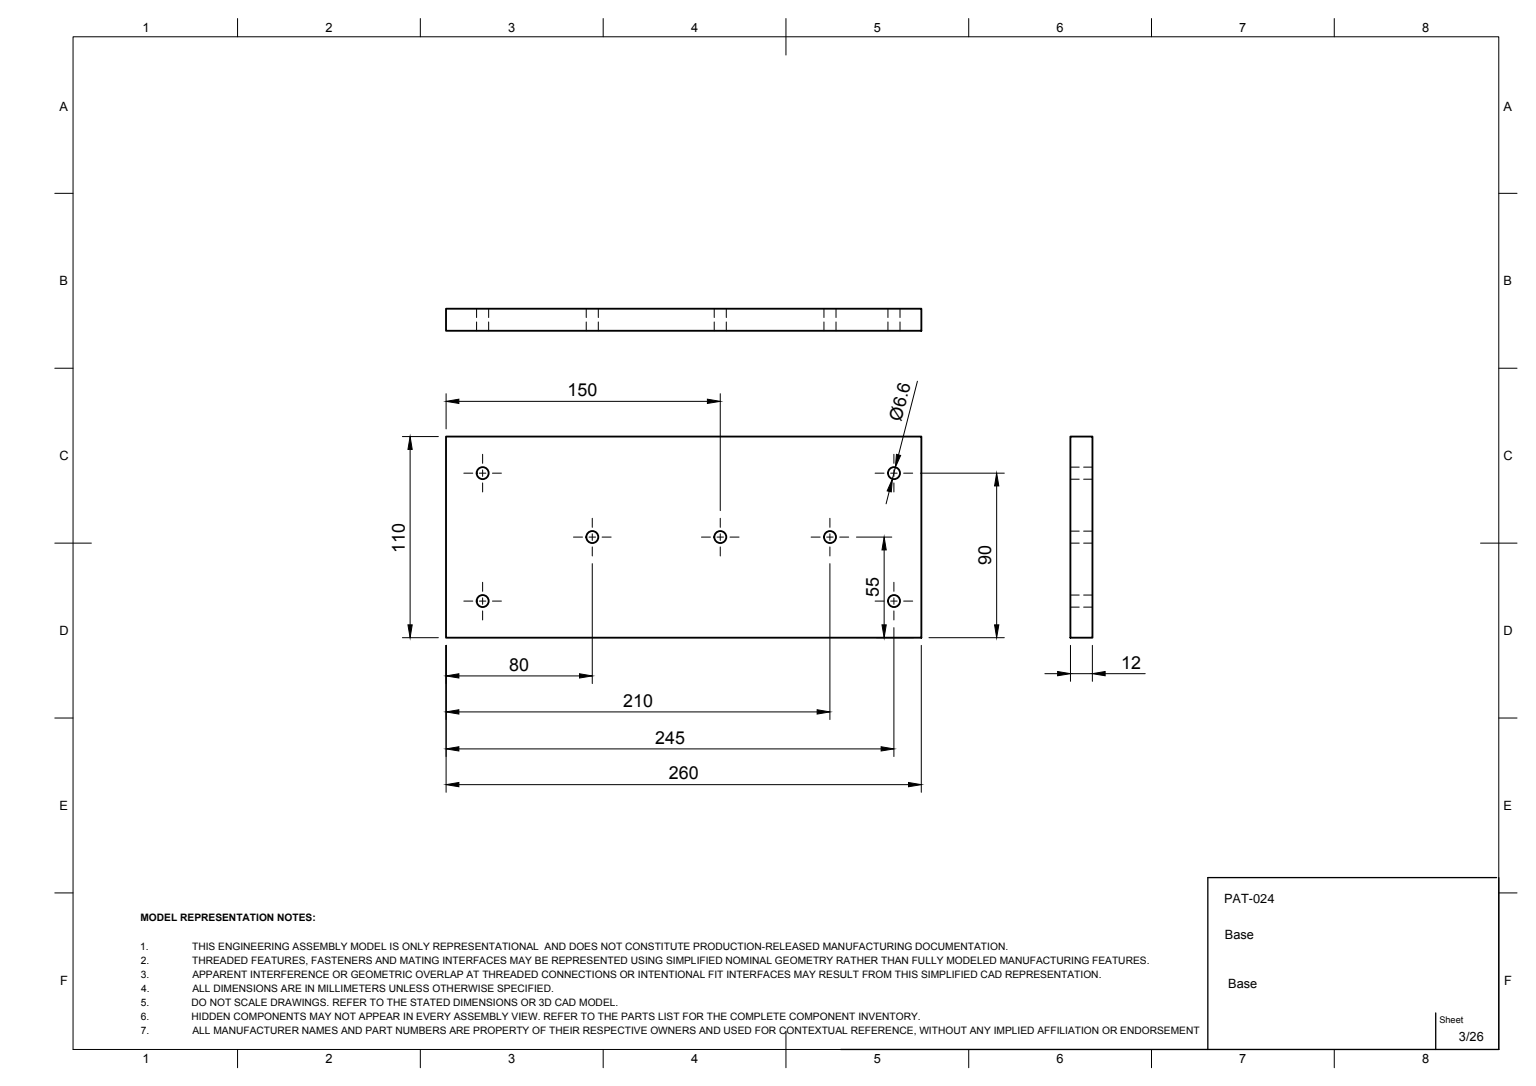
ISO-10303-21;
HEADER;
/* Generated by software containing ST-Developer
 * from STEP Tools, Inc. (www.steptools.com) 
 */

FILE_DESCRIPTION(
/* description */ ('Compact handwheel screw vise'),
/* implementation_level */ '2;1');

FILE_NAME(
/* name */ 'Base.step',
/* time_stamp */ '2026-10-29T16:08:22-07:00',
/* author */ (''),
/* organization */ (''),
/* preprocessor_version */ 'ST-DEVELOPER v20.2',
/* originating_system */ 'Autodesk Translation Framework v15.17.0.0',
/* authorisation */ '');

FILE_SCHEMA (('AUTOMOTIVE_DESIGN { 1 0 10303 214 3 1 1 }'));
ENDSEC;

DATA;
#10=MECHANICAL_DESIGN_GEOMETRIC_PRESENTATION_REPRESENTATION('',(#644),#25074);
#588=SHAPE_REPRESENTATION_RELATIONSHIP('SRR','None',#25196,#616);
#616=ADVANCED_BREP_SHAPE_REPRESENTATION('',(#680),#25043);
#644=STYLED_ITEM('',(#25418),#680);
#680=MANIFOLD_SOLID_BREP('Body1',#8052);
#712=FACE_BOUND('',#1494,.T.);
#713=FACE_BOUND('',#1495,.T.);
#714=FACE_BOUND('',#1496,.T.);
#715=FACE_BOUND('',#1497,.T.);
#716=FACE_BOUND('',#1498,.T.);
#717=FACE_BOUND('',#1499,.T.);
#718=FACE_BOUND('',#1500,.T.);
#719=FACE_BOUND('',#1502,.T.);
#720=FACE_BOUND('',#1503,.T.);
#721=FACE_BOUND('',#1504,.T.);
#722=FACE_BOUND('',#1505,.T.);
#723=FACE_BOUND('',#1506,.T.);
#724=FACE_BOUND('',#1507,.T.);
#725=FACE_BOUND('',#1508,.T.);
#822=PLANE('',#8425);
#823=PLANE('',#8426);
#824=PLANE('',#8427);
#825=PLANE('',#8428);
#826=PLANE('',#8429);
#827=PLANE('',#8430);
#1012=FACE_OUTER_BOUND('',#1482,.T.);
#1013=FACE_OUTER_BOUND('',#1483,.T.);
#1014=FACE_OUTER_BOUND('',#1484,.T.);
#1015=FACE_OUTER_BOUND('',#1485,.T.);
#1016=FACE_OUTER_BOUND('',#1486,.T.);
#1017=FACE_OUTER_BOUND('',#1487,.T.);
#1018=FACE_OUTER_BOUND('',#1488,.T.);
#1019=FACE_OUTER_BOUND('',#1489,.T.);
#1020=FACE_OUTER_BOUND('',#1490,.T.);
#1021=FACE_OUTER_BOUND('',#1491,.T.);
#1022=FACE_OUTER_BOUND('',#1492,.T.);
#1023=FACE_OUTER_BOUND('',#1493,.T.);
#1024=FACE_OUTER_BOUND('',#1501,.T.);
#1482=EDGE_LOOP('',(#5159,#5160,#5161,#5162));
#1483=EDGE_LOOP('',(#5163,#5164,#5165,#5166));
#1484=EDGE_LOOP('',(#5167,#5168,#5169,#5170));
#1485=EDGE_LOOP('',(#5171,#5172,#5173,#5174));
#1486=EDGE_LOOP('',(#5175,#5176,#5177,#5178));
#1487=EDGE_LOOP('',(#5179,#5180,#5181,#5182));
#1488=EDGE_LOOP('',(#5183,#5184,#5185,#5186));
#1489=EDGE_LOOP('',(#5187,#5188,#5189,#5190));
#1490=EDGE_LOOP('',(#5191,#5192,#5193,#5194));
#1491=EDGE_LOOP('',(#5195,#5196,#5197,#5198));
#1492=EDGE_LOOP('',(#5199,#5200,#5201,#5202));
#1493=EDGE_LOOP('',(#5203,#5204,#5205,#5206));
#1494=EDGE_LOOP('',(#5207));
#1495=EDGE_LOOP('',(#5208));
#1496=EDGE_LOOP('',(#5209));
#1497=EDGE_LOOP('',(#5210));
#1498=EDGE_LOOP('',(#5211));
#1499=EDGE_LOOP('',(#5212));
#1500=EDGE_LOOP('',(#5213));
#1501=EDGE_LOOP('',(#5214,#5215,#5216,#5217));
#1502=EDGE_LOOP('',(#5218));
#1503=EDGE_LOOP('',(#5219));
#1504=EDGE_LOOP('',(#5220));
#1505=EDGE_LOOP('',(#5221));
#1506=EDGE_LOOP('',(#5222));
#1507=EDGE_LOOP('',(#5223));
#1508=EDGE_LOOP('',(#5224));
#2062=LINE('',#11325,#2570);
#2063=LINE('',#11331,#2571);
#2064=LINE('',#11337,#2572);
#2065=LINE('',#11343,#2573);
#2066=LINE('',#11349,#2574);
#2067=LINE('',#11355,#2575);
#2068=LINE('',#11361,#2576);
#2069=LINE('',#11366,#2577);
#2070=LINE('',#11368,#2578);
#2071=LINE('',#11370,#2579);
#2072=LINE('',#11371,#2580);
#2073=LINE('',#11374,#2581);
#2074=LINE('',#11376,#2582);
#2075=LINE('',#11377,#2583);
#2076=LINE('',#11380,#2584);
#2077=LINE('',#11382,#2585);
#2078=LINE('',#11383,#2586);
#2079=LINE('',#11385,#2587);
#2080=LINE('',#11386,#2588);
#2570=VECTOR('',#9214,0.33);
#2571=VECTOR('',#9221,0.33);
#2572=VECTOR('',#9228,0.329999999999998);
#2573=VECTOR('',#9235,0.33);
#2574=VECTOR('',#9242,0.329999999999998);
#2575=VECTOR('',#9249,0.33);
#2576=VECTOR('',#9256,0.329999999999998);
#2577=VECTOR('',#9261,1.);
#2578=VECTOR('',#9262,1.);
#2579=VECTOR('',#9263,1.);
#2580=VECTOR('',#9264,1.);
#2581=VECTOR('',#9267,1.);
#2582=VECTOR('',#9268,1.);
#2583=VECTOR('',#9269,1.);
#2584=VECTOR('',#9272,1.);
#2585=VECTOR('',#9273,1.);
#2586=VECTOR('',#9274,1.);
#2587=VECTOR('',#9277,1.);
#2588=VECTOR('',#9278,1.);
#3078=CIRCLE('',#8405,0.33);
#3079=CIRCLE('',#8406,0.33);
#3080=CIRCLE('',#8408,0.33);
#3081=CIRCLE('',#8409,0.33);
#3082=CIRCLE('',#8411,0.329999999999998);
#3083=CIRCLE('',#8412,0.329999999999998);
#3084=CIRCLE('',#8414,0.33);
#3085=CIRCLE('',#8415,0.33);
#3086=CIRCLE('',#8417,0.329999999999998);
#3087=CIRCLE('',#8418,0.329999999999998);
#3088=CIRCLE('',#8420,0.33);
#3089=CIRCLE('',#8421,0.33);
#3090=CIRCLE('',#8423,0.329999999999998);
#3091=CIRCLE('',#8424,0.329999999999998);
#3333=VERTEX_POINT('',#11322);
#3334=VERTEX_POINT('',#11324);
#3335=VERTEX_POINT('',#11328);
#3336=VERTEX_POINT('',#11330);
#3337=VERTEX_POINT('',#11334);
#3338=VERTEX_POINT('',#11336);
#3339=VERTEX_POINT('',#11340);
#3340=VERTEX_POINT('',#11342);
#3341=VERTEX_POINT('',#11346);
#3342=VERTEX_POINT('',#11348);
#3343=VERTEX_POINT('',#11352);
#3344=VERTEX_POINT('',#11354);
#3345=VERTEX_POINT('',#11358);
#3346=VERTEX_POINT('',#11360);
#3347=VERTEX_POINT('',#11364);
#3348=VERTEX_POINT('',#11365);
#3349=VERTEX_POINT('',#11367);
#3350=VERTEX_POINT('',#11369);
#3351=VERTEX_POINT('',#11373);
#3352=VERTEX_POINT('',#11375);
#3353=VERTEX_POINT('',#11379);
#3354=VERTEX_POINT('',#11381);
#4066=EDGE_CURVE('',#3333,#3333,#3078,.T.);
#4067=EDGE_CURVE('',#3333,#3334,#2062,.T.);
#4068=EDGE_CURVE('',#3334,#3334,#3079,.T.);
#4069=EDGE_CURVE('',#3335,#3335,#3080,.T.);
#4070=EDGE_CURVE('',#3335,#3336,#2063,.T.);
#4071=EDGE_CURVE('',#3336,#3336,#3081,.T.);
#4072=EDGE_CURVE('',#3337,#3337,#3082,.T.);
#4073=EDGE_CURVE('',#3337,#3338,#2064,.T.);
#4074=EDGE_CURVE('',#3338,#3338,#3083,.T.);
#4075=EDGE_CURVE('',#3339,#3339,#3084,.T.);
#4076=EDGE_CURVE('',#3339,#3340,#2065,.T.);
#4077=EDGE_CURVE('',#3340,#3340,#3085,.T.);
#4078=EDGE_CURVE('',#3341,#3341,#3086,.T.);
#4079=EDGE_CURVE('',#3341,#3342,#2066,.T.);
#4080=EDGE_CURVE('',#3342,#3342,#3087,.T.);
#4081=EDGE_CURVE('',#3343,#3343,#3088,.T.);
#4082=EDGE_CURVE('',#3343,#3344,#2067,.T.);
#4083=EDGE_CURVE('',#3344,#3344,#3089,.T.);
#4084=EDGE_CURVE('',#3345,#3345,#3090,.T.);
#4085=EDGE_CURVE('',#3345,#3346,#2068,.T.);
#4086=EDGE_CURVE('',#3346,#3346,#3091,.T.);
#4087=EDGE_CURVE('',#3347,#3348,#2069,.T.);
#4088=EDGE_CURVE('',#3348,#3349,#2070,.T.);
#4089=EDGE_CURVE('',#3350,#3349,#2071,.T.);
#4090=EDGE_CURVE('',#3347,#3350,#2072,.T.);
#4091=EDGE_CURVE('',#3351,#3347,#2073,.T.);
#4092=EDGE_CURVE('',#3352,#3350,#2074,.T.);
#4093=EDGE_CURVE('',#3351,#3352,#2075,.T.);
#4094=EDGE_CURVE('',#3353,#3351,#2076,.T.);
#4095=EDGE_CURVE('',#3354,#3352,#2077,.T.);
#4096=EDGE_CURVE('',#3353,#3354,#2078,.T.);
#4097=EDGE_CURVE('',#3348,#3353,#2079,.T.);
#4098=EDGE_CURVE('',#3349,#3354,#2080,.T.);
#5159=ORIENTED_EDGE('',*,*,#4066,.F.);
#5160=ORIENTED_EDGE('',*,*,#4067,.T.);
#5161=ORIENTED_EDGE('',*,*,#4068,.F.);
#5162=ORIENTED_EDGE('',*,*,#4067,.F.);
#5163=ORIENTED_EDGE('',*,*,#4069,.F.);
#5164=ORIENTED_EDGE('',*,*,#4070,.T.);
#5165=ORIENTED_EDGE('',*,*,#4071,.F.);
#5166=ORIENTED_EDGE('',*,*,#4070,.F.);
#5167=ORIENTED_EDGE('',*,*,#4072,.F.);
#5168=ORIENTED_EDGE('',*,*,#4073,.T.);
#5169=ORIENTED_EDGE('',*,*,#4074,.F.);
#5170=ORIENTED_EDGE('',*,*,#4073,.F.);
#5171=ORIENTED_EDGE('',*,*,#4075,.F.);
#5172=ORIENTED_EDGE('',*,*,#4076,.T.);
#5173=ORIENTED_EDGE('',*,*,#4077,.F.);
#5174=ORIENTED_EDGE('',*,*,#4076,.F.);
#5175=ORIENTED_EDGE('',*,*,#4078,.F.);
#5176=ORIENTED_EDGE('',*,*,#4079,.T.);
#5177=ORIENTED_EDGE('',*,*,#4080,.F.);
#5178=ORIENTED_EDGE('',*,*,#4079,.F.);
#5179=ORIENTED_EDGE('',*,*,#4081,.F.);
#5180=ORIENTED_EDGE('',*,*,#4082,.T.);
#5181=ORIENTED_EDGE('',*,*,#4083,.F.);
#5182=ORIENTED_EDGE('',*,*,#4082,.F.);
#5183=ORIENTED_EDGE('',*,*,#4084,.F.);
#5184=ORIENTED_EDGE('',*,*,#4085,.T.);
#5185=ORIENTED_EDGE('',*,*,#4086,.F.);
#5186=ORIENTED_EDGE('',*,*,#4085,.F.);
#5187=ORIENTED_EDGE('',*,*,#4087,.T.);
#5188=ORIENTED_EDGE('',*,*,#4088,.T.);
#5189=ORIENTED_EDGE('',*,*,#4089,.F.);
#5190=ORIENTED_EDGE('',*,*,#4090,.F.);
#5191=ORIENTED_EDGE('',*,*,#4091,.T.);
#5192=ORIENTED_EDGE('',*,*,#4090,.T.);
#5193=ORIENTED_EDGE('',*,*,#4092,.F.);
#5194=ORIENTED_EDGE('',*,*,#4093,.F.);
#5195=ORIENTED_EDGE('',*,*,#4094,.T.);
#5196=ORIENTED_EDGE('',*,*,#4093,.T.);
#5197=ORIENTED_EDGE('',*,*,#4095,.F.);
#5198=ORIENTED_EDGE('',*,*,#4096,.F.);
#5199=ORIENTED_EDGE('',*,*,#4097,.T.);
#5200=ORIENTED_EDGE('',*,*,#4096,.T.);
#5201=ORIENTED_EDGE('',*,*,#4098,.F.);
#5202=ORIENTED_EDGE('',*,*,#4088,.F.);
#5203=ORIENTED_EDGE('',*,*,#4098,.T.);
#5204=ORIENTED_EDGE('',*,*,#4095,.T.);
#5205=ORIENTED_EDGE('',*,*,#4092,.T.);
#5206=ORIENTED_EDGE('',*,*,#4089,.T.);
#5207=ORIENTED_EDGE('',*,*,#4086,.T.);
#5208=ORIENTED_EDGE('',*,*,#4083,.T.);
#5209=ORIENTED_EDGE('',*,*,#4080,.T.);
#5210=ORIENTED_EDGE('',*,*,#4077,.T.);
#5211=ORIENTED_EDGE('',*,*,#4074,.T.);
#5212=ORIENTED_EDGE('',*,*,#4071,.T.);
#5213=ORIENTED_EDGE('',*,*,#4068,.T.);
#5214=ORIENTED_EDGE('',*,*,#4097,.F.);
#5215=ORIENTED_EDGE('',*,*,#4087,.F.);
#5216=ORIENTED_EDGE('',*,*,#4091,.F.);
#5217=ORIENTED_EDGE('',*,*,#4094,.F.);
#5218=ORIENTED_EDGE('',*,*,#4084,.T.);
#5219=ORIENTED_EDGE('',*,*,#4081,.T.);
#5220=ORIENTED_EDGE('',*,*,#4078,.T.);
#5221=ORIENTED_EDGE('',*,*,#4075,.T.);
#5222=ORIENTED_EDGE('',*,*,#4072,.T.);
#5223=ORIENTED_EDGE('',*,*,#4069,.T.);
#5224=ORIENTED_EDGE('',*,*,#4066,.T.);
#7345=CYLINDRICAL_SURFACE('',#8404,0.33);
#7346=CYLINDRICAL_SURFACE('',#8407,0.33);
#7347=CYLINDRICAL_SURFACE('',#8410,0.329999999999998);
#7348=CYLINDRICAL_SURFACE('',#8413,0.33);
#7349=CYLINDRICAL_SURFACE('',#8416,0.329999999999998);
#7350=CYLINDRICAL_SURFACE('',#8419,0.33);
#7351=CYLINDRICAL_SURFACE('',#8422,0.329999999999998);
#7582=ADVANCED_FACE('',(#1012),#7345,.F.);
#7583=ADVANCED_FACE('',(#1013),#7346,.F.);
#7584=ADVANCED_FACE('',(#1014),#7347,.F.);
#7585=ADVANCED_FACE('',(#1015),#7348,.F.);
#7586=ADVANCED_FACE('',(#1016),#7349,.F.);
#7587=ADVANCED_FACE('',(#1017),#7350,.F.);
#7588=ADVANCED_FACE('',(#1018),#7351,.F.);
#7589=ADVANCED_FACE('',(#1019),#822,.T.);
#7590=ADVANCED_FACE('',(#1020),#823,.T.);
#7591=ADVANCED_FACE('',(#1021),#824,.T.);
#7592=ADVANCED_FACE('',(#1022),#825,.T.);
#7593=ADVANCED_FACE('',(#1023,#712,#713,#714,#715,#716,#717,#718),#826,
 .T.);
#7594=ADVANCED_FACE('',(#1024,#719,#720,#721,#722,#723,#724,#725),#827,
 .F.);
#8052=CLOSED_SHELL('',(#7582,#7583,#7584,#7585,#7586,#7587,#7588,#7589,
#7590,#7591,#7592,#7593,#7594));
#8403=AXIS2_PLACEMENT_3D('',#11320,#9208,#9209);
#8404=AXIS2_PLACEMENT_3D('',#11321,#9210,#9211);
#8405=AXIS2_PLACEMENT_3D('',#11323,#9212,#9213);
#8406=AXIS2_PLACEMENT_3D('',#11326,#9215,#9216);
#8407=AXIS2_PLACEMENT_3D('',#11327,#9217,#9218);
#8408=AXIS2_PLACEMENT_3D('',#11329,#9219,#9220);
#8409=AXIS2_PLACEMENT_3D('',#11332,#9222,#9223);
#8410=AXIS2_PLACEMENT_3D('',#11333,#9224,#9225);
#8411=AXIS2_PLACEMENT_3D('',#11335,#9226,#9227);
#8412=AXIS2_PLACEMENT_3D('',#11338,#9229,#9230);
#8413=AXIS2_PLACEMENT_3D('',#11339,#9231,#9232);
#8414=AXIS2_PLACEMENT_3D('',#11341,#9233,#9234);
#8415=AXIS2_PLACEMENT_3D('',#11344,#9236,#9237);
#8416=AXIS2_PLACEMENT_3D('',#11345,#9238,#9239);
#8417=AXIS2_PLACEMENT_3D('',#11347,#9240,#9241);
#8418=AXIS2_PLACEMENT_3D('',#11350,#9243,#9244);
#8419=AXIS2_PLACEMENT_3D('',#11351,#9245,#9246);
#8420=AXIS2_PLACEMENT_3D('',#11353,#9247,#9248);
#8421=AXIS2_PLACEMENT_3D('',#11356,#9250,#9251);
#8422=AXIS2_PLACEMENT_3D('',#11357,#9252,#9253);
#8423=AXIS2_PLACEMENT_3D('',#11359,#9254,#9255);
#8424=AXIS2_PLACEMENT_3D('',#11362,#9257,#9258);
#8425=AXIS2_PLACEMENT_3D('',#11363,#9259,#9260);
#8426=AXIS2_PLACEMENT_3D('',#11372,#9265,#9266);
#8427=AXIS2_PLACEMENT_3D('',#11378,#9270,#9271);
#8428=AXIS2_PLACEMENT_3D('',#11384,#9275,#9276);
#8429=AXIS2_PLACEMENT_3D('',#11387,#9279,#9280);
#8430=AXIS2_PLACEMENT_3D('',#11388,#9281,#9282);
#9208=DIRECTION('axis',(0.,0.,1.));
#9209=DIRECTION('refdir',(1.,0.,0.));
#9210=DIRECTION('center_axis',(0.,0.,1.));
#9211=DIRECTION('ref_axis',(1.,0.,0.));
#9212=DIRECTION('center_axis',(0.,0.,1.));
#9213=DIRECTION('ref_axis',(1.,0.,0.));
#9214=DIRECTION('',(0.,0.,1.));
#9215=DIRECTION('center_axis',(0.,0.,-1.));
#9216=DIRECTION('ref_axis',(1.,0.,0.));
#9217=DIRECTION('center_axis',(0.,0.,1.));
#9218=DIRECTION('ref_axis',(1.,0.,0.));
#9219=DIRECTION('center_axis',(0.,0.,1.));
#9220=DIRECTION('ref_axis',(1.,0.,0.));
#9221=DIRECTION('',(0.,0.,1.));
#9222=DIRECTION('center_axis',(0.,0.,-1.));
#9223=DIRECTION('ref_axis',(1.,0.,0.));
#9224=DIRECTION('center_axis',(0.,0.,1.));
#9225=DIRECTION('ref_axis',(1.,0.,0.));
#9226=DIRECTION('center_axis',(0.,0.,1.));
#9227=DIRECTION('ref_axis',(1.,0.,0.));
#9228=DIRECTION('',(0.,0.,1.));
#9229=DIRECTION('center_axis',(0.,0.,-1.));
#9230=DIRECTION('ref_axis',(1.,0.,0.));
#9231=DIRECTION('center_axis',(0.,0.,1.));
#9232=DIRECTION('ref_axis',(1.,0.,0.));
#9233=DIRECTION('center_axis',(0.,0.,1.));
#9234=DIRECTION('ref_axis',(1.,0.,0.));
#9235=DIRECTION('',(0.,0.,1.));
#9236=DIRECTION('center_axis',(0.,0.,-1.));
#9237=DIRECTION('ref_axis',(1.,0.,0.));
#9238=DIRECTION('center_axis',(0.,0.,1.));
#9239=DIRECTION('ref_axis',(1.,0.,0.));
#9240=DIRECTION('center_axis',(0.,0.,1.));
#9241=DIRECTION('ref_axis',(1.,0.,0.));
#9242=DIRECTION('',(0.,0.,1.));
#9243=DIRECTION('center_axis',(0.,0.,-1.));
#9244=DIRECTION('ref_axis',(1.,0.,0.));
#9245=DIRECTION('center_axis',(0.,0.,1.));
#9246=DIRECTION('ref_axis',(1.,0.,0.));
#9247=DIRECTION('center_axis',(0.,0.,1.));
#9248=DIRECTION('ref_axis',(1.,0.,0.));
#9249=DIRECTION('',(0.,0.,1.));
#9250=DIRECTION('center_axis',(0.,0.,-1.));
#9251=DIRECTION('ref_axis',(1.,0.,0.));
#9252=DIRECTION('center_axis',(0.,0.,1.));
#9253=DIRECTION('ref_axis',(1.,0.,0.));
#9254=DIRECTION('center_axis',(0.,0.,1.));
#9255=DIRECTION('ref_axis',(1.,0.,0.));
#9256=DIRECTION('',(0.,0.,1.));
#9257=DIRECTION('center_axis',(0.,0.,-1.));
#9258=DIRECTION('ref_axis',(1.,0.,0.));
#9259=DIRECTION('center_axis',(0.,1.,0.));
#9260=DIRECTION('ref_axis',(-1.,0.,0.));
#9261=DIRECTION('',(-1.,0.,0.));
#9262=DIRECTION('',(0.,0.,1.));
#9263=DIRECTION('',(-1.,0.,0.));
#9264=DIRECTION('',(0.,0.,1.));
#9265=DIRECTION('center_axis',(1.,0.,0.));
#9266=DIRECTION('ref_axis',(0.,1.,0.));
#9267=DIRECTION('',(0.,1.,0.));
#9268=DIRECTION('',(0.,1.,0.));
#9269=DIRECTION('',(0.,0.,1.));
#9270=DIRECTION('center_axis',(0.,-1.,0.));
#9271=DIRECTION('ref_axis',(1.,0.,0.));
#9272=DIRECTION('',(1.,0.,0.));
#9273=DIRECTION('',(1.,0.,0.));
#9274=DIRECTION('',(0.,0.,1.));
#9275=DIRECTION('center_axis',(-1.,0.,0.));
#9276=DIRECTION('ref_axis',(0.,-1.,0.));
#9277=DIRECTION('',(0.,-1.,0.));
#9278=DIRECTION('',(0.,-1.,0.));
#9279=DIRECTION('center_axis',(0.,0.,1.));
#9280=DIRECTION('ref_axis',(1.,0.,0.));
#9281=DIRECTION('center_axis',(0.,0.,1.));
#9282=DIRECTION('ref_axis',(1.,0.,0.));
#11320=CARTESIAN_POINT('',(0.,0.,0.));
#11321=CARTESIAN_POINT('Origin',(11.,0.,-0.1));
#11322=CARTESIAN_POINT('',(10.67,-4.04133443718627E-17,0.));
#11323=CARTESIAN_POINT('Origin',(11.,0.,0.));
#11324=CARTESIAN_POINT('',(10.67,4.04133443718627E-17,1.2));
#11325=CARTESIAN_POINT('',(10.67,-4.04133443718627E-17,-0.1));
#11326=CARTESIAN_POINT('Origin',(11.,0.,1.2));
#11327=CARTESIAN_POINT('Origin',(1.5,-3.5,-0.1));
#11328=CARTESIAN_POINT('',(1.17,-3.5,0.));
#11329=CARTESIAN_POINT('Origin',(1.5,-3.5,0.));
#11330=CARTESIAN_POINT('',(1.17,-3.5,1.2));
#11331=CARTESIAN_POINT('',(1.17,-3.5,-0.1));
#11332=CARTESIAN_POINT('Origin',(1.5,-3.5,1.2));
#11333=CARTESIAN_POINT('Origin',(24.,-3.5,-0.1));
#11334=CARTESIAN_POINT('',(23.67,-3.5,0.));
#11335=CARTESIAN_POINT('Origin',(24.,-3.5,0.));
#11336=CARTESIAN_POINT('',(23.67,-3.5,1.2));
#11337=CARTESIAN_POINT('',(23.67,-3.5,-0.1));
#11338=CARTESIAN_POINT('Origin',(24.,-3.5,1.2));
#11339=CARTESIAN_POINT('Origin',(1.5,3.5,-0.1));
#11340=CARTESIAN_POINT('',(1.17,3.5,0.));
#11341=CARTESIAN_POINT('Origin',(1.5,3.5,0.));
#11342=CARTESIAN_POINT('',(1.17,3.5,1.2));
#11343=CARTESIAN_POINT('',(1.17,3.5,-0.1));
#11344=CARTESIAN_POINT('Origin',(1.5,3.5,1.2));
#11345=CARTESIAN_POINT('Origin',(24.,3.5,-0.1));
#11346=CARTESIAN_POINT('',(23.67,3.5,0.));
#11347=CARTESIAN_POINT('Origin',(24.,3.5,0.));
#11348=CARTESIAN_POINT('',(23.67,3.5,1.2));
#11349=CARTESIAN_POINT('',(23.67,3.5,-0.1));
#11350=CARTESIAN_POINT('Origin',(24.,3.5,1.2));
#11351=CARTESIAN_POINT('Origin',(5.,0.,-0.1));
#11352=CARTESIAN_POINT('',(4.67,-4.04133443718627E-17,0.));
#11353=CARTESIAN_POINT('Origin',(5.,0.,0.));
#11354=CARTESIAN_POINT('',(4.67,4.04133443718627E-17,1.2));
#11355=CARTESIAN_POINT('',(4.67,-4.04133443718627E-17,-0.1));
#11356=CARTESIAN_POINT('Origin',(5.,0.,1.2));
#11357=CARTESIAN_POINT('Origin',(18.,0.,-0.1));
#11358=CARTESIAN_POINT('',(17.67,-4.04133443718624E-17,0.));
#11359=CARTESIAN_POINT('Origin',(18.,0.,0.));
#11360=CARTESIAN_POINT('',(17.67,4.04133443718624E-17,1.2));
#11361=CARTESIAN_POINT('',(17.67,-4.04133443718624E-17,-0.1));
#11362=CARTESIAN_POINT('Origin',(18.,0.,1.2));
#11363=CARTESIAN_POINT('Origin',(26.,5.5,0.));
#11364=CARTESIAN_POINT('',(26.,5.5,0.));
#11365=CARTESIAN_POINT('',(0.,5.5,0.));
#11366=CARTESIAN_POINT('',(26.,5.5,0.));
#11367=CARTESIAN_POINT('',(0.,5.5,1.2));
#11368=CARTESIAN_POINT('',(0.,5.5,0.));
#11369=CARTESIAN_POINT('',(26.,5.5,1.2));
#11370=CARTESIAN_POINT('',(26.,5.5,1.2));
#11371=CARTESIAN_POINT('',(26.,5.5,0.));
#11372=CARTESIAN_POINT('Origin',(26.,-5.5,0.));
#11373=CARTESIAN_POINT('',(26.,-5.5,0.));
#11374=CARTESIAN_POINT('',(26.,-5.5,0.));
#11375=CARTESIAN_POINT('',(26.,-5.5,1.2));
#11376=CARTESIAN_POINT('',(26.,-5.5,1.2));
#11377=CARTESIAN_POINT('',(26.,-5.5,0.));
#11378=CARTESIAN_POINT('Origin',(0.,-5.5,0.));
#11379=CARTESIAN_POINT('',(0.,-5.5,0.));
#11380=CARTESIAN_POINT('',(0.,-5.5,0.));
#11381=CARTESIAN_POINT('',(0.,-5.5,1.2));
#11382=CARTESIAN_POINT('',(0.,-5.5,1.2));
#11383=CARTESIAN_POINT('',(0.,-5.5,0.));
#11384=CARTESIAN_POINT('Origin',(0.,5.5,0.));
#11385=CARTESIAN_POINT('',(0.,5.5,0.));
#11386=CARTESIAN_POINT('',(0.,5.5,1.2));
#11387=CARTESIAN_POINT('Origin',(13.,0.,1.2));
#11388=CARTESIAN_POINT('Origin',(13.,0.,0.));
#25009=UNCERTAINTY_MEASURE_WITH_UNIT(LENGTH_MEASURE(0.001),#25075,
'DISTANCE_ACCURACY_VALUE',
'Maximum model space distance between geometric entities at asserted c
onnectivities');
#25040=UNCERTAINTY_MEASURE_WITH_UNIT(LENGTH_MEASURE(0.001),#25075,
'DISTANCE_ACCURACY_VALUE',
'Maximum model space distance between geometric entities at asserted c
onnectivities');
#25043=(
GEOMETRIC_REPRESENTATION_CONTEXT(3)
GLOBAL_UNCERTAINTY_ASSIGNED_CONTEXT((#25009))
GLOBAL_UNIT_ASSIGNED_CONTEXT((#25075,#25077,#25078))
REPRESENTATION_CONTEXT('','3D')
);
#25074=(
GEOMETRIC_REPRESENTATION_CONTEXT(3)
GLOBAL_UNCERTAINTY_ASSIGNED_CONTEXT((#25040))
GLOBAL_UNIT_ASSIGNED_CONTEXT((#25075,#25077,#25078))
REPRESENTATION_CONTEXT('','3D')
);
#25075=(
LENGTH_UNIT()
NAMED_UNIT(*)
SI_UNIT(.CENTI.,.METRE.)
);
#25077=(
NAMED_UNIT(*)
PLANE_ANGLE_UNIT()
SI_UNIT($,.RADIAN.)
);
#25078=(
NAMED_UNIT(*)
SI_UNIT($,.STERADIAN.)
SOLID_ANGLE_UNIT()
);
#25081=SHAPE_DEFINITION_REPRESENTATION(#25114,#25196);
#25114=PRODUCT_DEFINITION_SHAPE('',$,#25230);
#25196=SHAPE_REPRESENTATION('',(#8403),#25043);
#25227=PRODUCT_DEFINITION_CONTEXT('part definition',#25328,'design');
#25230=PRODUCT_DEFINITION('Base','Base',#25263,#25227);
#25263=PRODUCT_DEFINITION_FORMATION('',$,#25332);
#25328=APPLICATION_CONTEXT(
'Core Data for Automotive Mechanical Design Process');
#25329=PRODUCT_CONTEXT('part definition',#25328,'mechanical');
#25332=PRODUCT('Base','Base','Base',(#25329));
#25412=COLOUR_RGB('Dark Blue',0.08,0.2,0.34);
#25413=FILL_AREA_STYLE_COLOUR('',#25412);
#25414=FILL_AREA_STYLE('',(#25413));
#25415=SURFACE_STYLE_FILL_AREA(#25414);
#25416=SURFACE_SIDE_STYLE('',(#25415));
#25417=SURFACE_STYLE_USAGE(.BOTH.,#25416);
#25418=PRESENTATION_STYLE_ASSIGNMENT((#25417));
ENDSEC;
END-ISO-10303-21;
